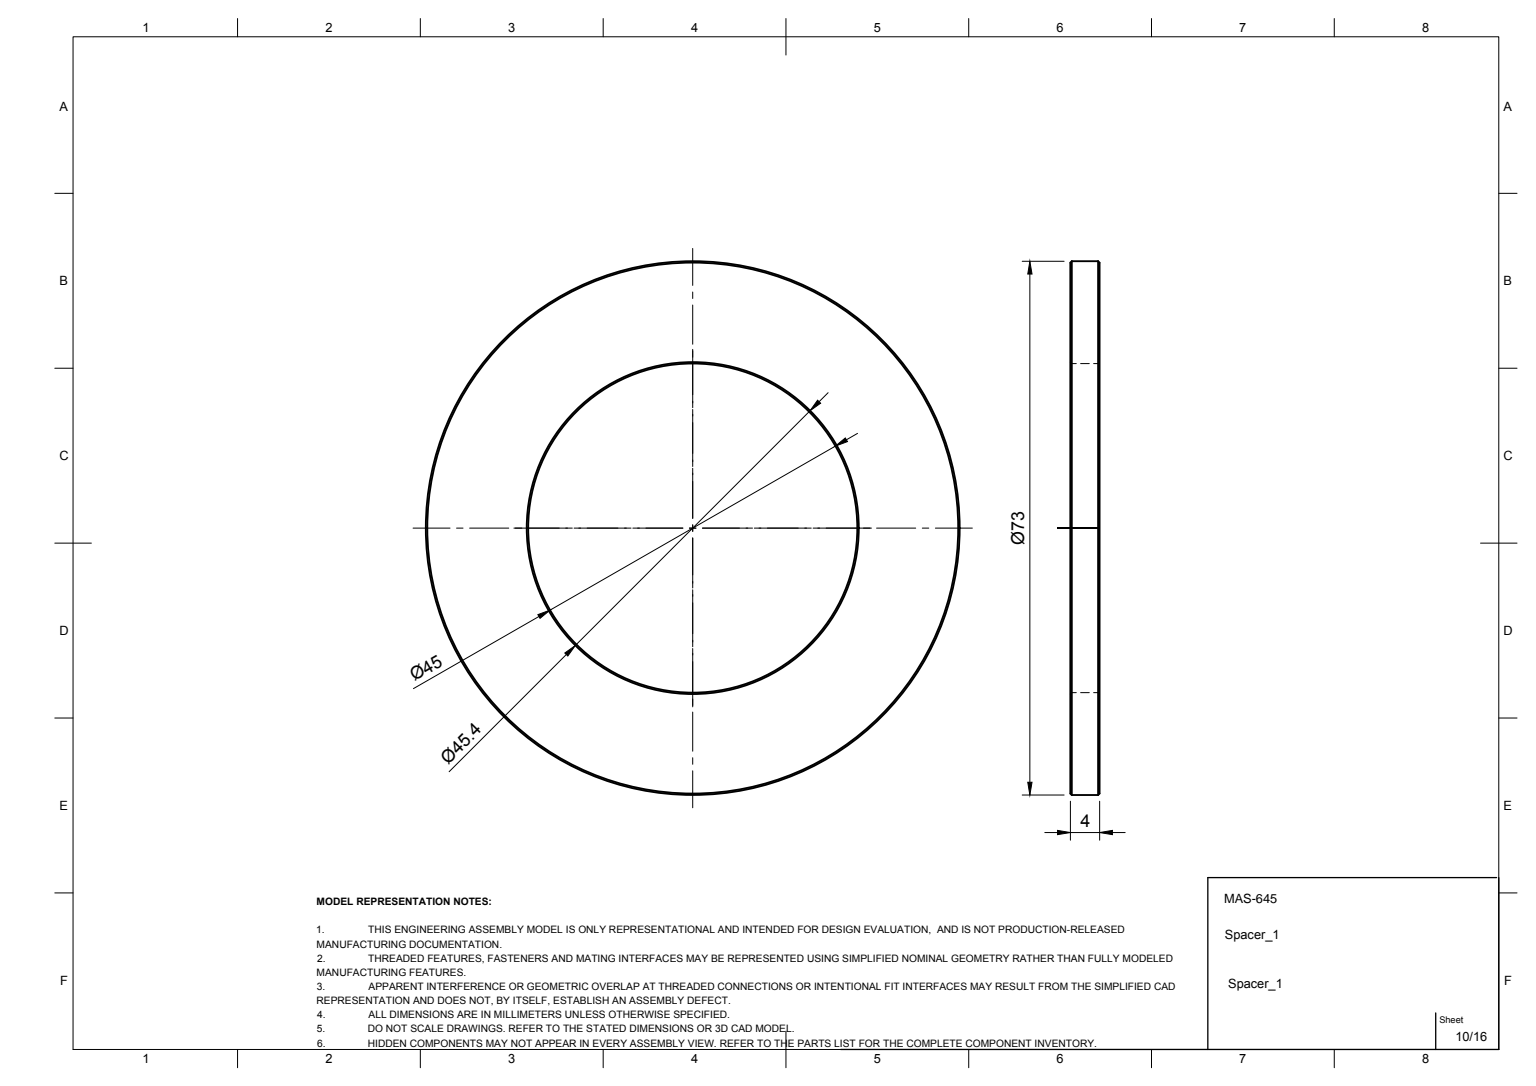
ISO-10303-21;
HEADER;
FILE_DESCRIPTION((''),'2;1');
FILE_NAME('Spacer_1.step','2026-10-09T10:54:55-07:00',(''),(''),'','','');
FILE_SCHEMA (('AUTOMOTIVE_DESIGN { 1 0 10303 214 3 1 1 }'));
ENDSEC;
DATA;
#10=MECHANICAL_DESIGN_GEOMETRIC_PRESENTATION_REPRESENTATION('',(#607),#63824);
#577=SHAPE_REPRESENTATION_RELATIONSHIP('SRR','None',#63891,#592) ;
#592=ADVANCED_BREP_SHAPE_REPRESENTATION('',(#622),#63821) ;
#607=STYLED_ITEM('',(#63963),#622) ;
#622=MANIFOLD_SOLID_BREP('Body1',#15506) ;
#794=FACE_BOUND('',#3406,.T.) ;
#795=FACE_BOUND('',#3412,.T.) ;
#1110=PLANE('',#17806) ;
#1111=PLANE('',#17816) ;
#1523=CYLINDRICAL_SURFACE('',#17808,36.5) ;
#1524=CYLINDRICAL_SURFACE('',#17812,22.5) ;
#2374=FACE_OUTER_BOUND('',#3404,.T.) ;
#2375=FACE_OUTER_BOUND('',#3405,.T.) ;
#2376=FACE_OUTER_BOUND('',#3407,.T.) ;
#2377=FACE_OUTER_BOUND('',#3408,.T.) ;
#2378=FACE_OUTER_BOUND('',#3409,.T.) ;
#2379=FACE_OUTER_BOUND('',#3410,.T.) ;
#2380=FACE_OUTER_BOUND('',#3411,.T.) ;
#2381=FACE_OUTER_BOUND('',#3413,.T.) ;
#3404=EDGE_LOOP('',(#14348,#14349,#14350,#14351)) ;
#3405=EDGE_LOOP('',(#14352)) ;
#3406=EDGE_LOOP('',(#14353)) ;
#3407=EDGE_LOOP('',(#14354,#14355,#14356,#14357)) ;
#3408=EDGE_LOOP('',(#14358,#14359,#14360,#14361)) ;
#3409=EDGE_LOOP('',(#14362,#14363,#14364,#14365)) ;
#3410=EDGE_LOOP('',(#14366,#14367,#14368,#14369)) ;
#3411=EDGE_LOOP('',(#14370)) ;
#3412=EDGE_LOOP('',(#14371)) ;
#3413=EDGE_LOOP('',(#14372,#14373,#14374,#14375)) ;
#4642=CIRCLE('',#17804,36.5) ;
#4643=CIRCLE('',#17805,36.3) ;
#4644=CIRCLE('',#17807,22.7) ;
#4645=CIRCLE('',#17809,36.5) ;
#4646=CIRCLE('',#17811,22.5) ;
#4647=CIRCLE('',#17813,22.5) ;
#4648=CIRCLE('',#17815,36.3) ;
#4649=CIRCLE('',#17817,22.7) ;
#5320=LINE('',#63622,#5976) ;
#5321=LINE('',#63630,#5977) ;
#5322=LINE('',#63634,#5978) ;
#5323=LINE('',#63637,#5979) ;
#5324=LINE('',#63641,#5980) ;
#5325=LINE('',#63647,#5981) ;
#5976=VECTOR('',#22792,36.4) ;
#5977=VECTOR('',#22803,36.5) ;
#5978=VECTOR('',#22808,22.6) ;
#5979=VECTOR('',#22811,22.5) ;
#5980=VECTOR('',#22816,36.4) ;
#5981=VECTOR('',#22825,22.6) ;
#7407=VERTEX_POINT('',#63619) ;
#7408=VERTEX_POINT('',#63621) ;
#7409=VERTEX_POINT('',#63625) ;
#7410=VERTEX_POINT('',#63628) ;
#7411=VERTEX_POINT('',#63632) ;
#7412=VERTEX_POINT('',#63636) ;
#7413=VERTEX_POINT('',#63640) ;
#7414=VERTEX_POINT('',#63644) ;
#9728=EDGE_CURVE('',#7407,#7407,#4642,.T.) ;
#9729=EDGE_CURVE('',#7407,#7408,#5320,.T.) ;
#9730=EDGE_CURVE('',#7408,#7408,#4643,.T.) ;
#9731=EDGE_CURVE('',#7409,#7409,#4644,.T.) ;
#9732=EDGE_CURVE('',#7410,#7410,#4645,.T.) ;
#9733=EDGE_CURVE('',#7410,#7407,#5321,.T.) ;
#9734=EDGE_CURVE('',#7411,#7411,#4646,.T.) ;
#9735=EDGE_CURVE('',#7411,#7409,#5322,.T.) ;
#9736=EDGE_CURVE('',#7411,#7412,#5323,.T.) ;
#9737=EDGE_CURVE('',#7412,#7412,#4647,.T.) ;
#9738=EDGE_CURVE('',#7410,#7413,#5324,.T.) ;
#9739=EDGE_CURVE('',#7413,#7413,#4648,.T.) ;
#9740=EDGE_CURVE('',#7414,#7414,#4649,.T.) ;
#9741=EDGE_CURVE('',#7412,#7414,#5325,.T.) ;
#14348=ORIENTED_EDGE('',*,*,#9728,.T.) ;
#14349=ORIENTED_EDGE('',*,*,#9729,.T.) ;
#14350=ORIENTED_EDGE('',*,*,#9730,.T.) ;
#14351=ORIENTED_EDGE('',*,*,#9729,.F.) ;
#14352=ORIENTED_EDGE('',*,*,#9730,.F.) ;
#14353=ORIENTED_EDGE('',*,*,#9731,.F.) ;
#14354=ORIENTED_EDGE('',*,*,#9732,.F.) ;
#14355=ORIENTED_EDGE('',*,*,#9733,.T.) ;
#14356=ORIENTED_EDGE('',*,*,#9728,.F.) ;
#14357=ORIENTED_EDGE('',*,*,#9733,.F.) ;
#14358=ORIENTED_EDGE('',*,*,#9734,.T.) ;
#14359=ORIENTED_EDGE('',*,*,#9735,.T.) ;
#14360=ORIENTED_EDGE('',*,*,#9731,.T.) ;
#14361=ORIENTED_EDGE('',*,*,#9735,.F.) ;
#14362=ORIENTED_EDGE('',*,*,#9734,.F.) ;
#14363=ORIENTED_EDGE('',*,*,#9736,.T.) ;
#14364=ORIENTED_EDGE('',*,*,#9737,.F.) ;
#14365=ORIENTED_EDGE('',*,*,#9736,.F.) ;
#14366=ORIENTED_EDGE('',*,*,#9732,.T.) ;
#14367=ORIENTED_EDGE('',*,*,#9738,.T.) ;
#14368=ORIENTED_EDGE('',*,*,#9739,.T.) ;
#14369=ORIENTED_EDGE('',*,*,#9738,.F.) ;
#14370=ORIENTED_EDGE('',*,*,#9739,.F.) ;
#14371=ORIENTED_EDGE('',*,*,#9740,.F.) ;
#14372=ORIENTED_EDGE('',*,*,#9737,.T.) ;
#14373=ORIENTED_EDGE('',*,*,#9741,.T.) ;
#14374=ORIENTED_EDGE('',*,*,#9740,.T.) ;
#14375=ORIENTED_EDGE('',*,*,#9741,.F.) ;
#14629=CONICAL_SURFACE('',#17803,36.4,0.785398163397449) ;
#14630=CONICAL_SURFACE('',#17810,22.6,0.785398163397449) ;
#14631=CONICAL_SURFACE('',#17814,36.4,0.785398163397448) ;
#14632=CONICAL_SURFACE('',#17818,22.6,0.785398163397448) ;
#15462=ADVANCED_FACE('',(#2374),#14629,.T.) ;
#15463=ADVANCED_FACE('',(#2375,#794),#1110,.F.) ;
#15464=ADVANCED_FACE('',(#2376),#1523,.T.) ;
#15465=ADVANCED_FACE('',(#2377),#14630,.F.) ;
#15466=ADVANCED_FACE('',(#2378),#1524,.F.) ;
#15467=ADVANCED_FACE('',(#2379),#14631,.T.) ;
#15468=ADVANCED_FACE('',(#2380,#795),#1111,.T.) ;
#15469=ADVANCED_FACE('',(#2381),#14632,.F.) ;
#15506=CLOSED_SHELL('',(#15462,#15463,#15464,#15465,#15466,#15467,#15468,
#15469)) ;
#17802=AXIS2_PLACEMENT_3D('',#63617,#22786,#22787) ;
#17803=AXIS2_PLACEMENT_3D('',#63618,#22788,#22789) ;
#17804=AXIS2_PLACEMENT_3D('',#63620,#22790,#22791) ;
#17805=AXIS2_PLACEMENT_3D('',#63623,#22793,#22794) ;
#17806=AXIS2_PLACEMENT_3D('',#63624,#22795,#22796) ;
#17807=AXIS2_PLACEMENT_3D('',#63626,#22797,#22798) ;
#17808=AXIS2_PLACEMENT_3D('',#63627,#22799,#22800) ;
#17809=AXIS2_PLACEMENT_3D('',#63629,#22801,#22802) ;
#17810=AXIS2_PLACEMENT_3D('',#63631,#22804,#22805) ;
#17811=AXIS2_PLACEMENT_3D('',#63633,#22806,#22807) ;
#17812=AXIS2_PLACEMENT_3D('',#63635,#22809,#22810) ;
#17813=AXIS2_PLACEMENT_3D('',#63638,#22812,#22813) ;
#17814=AXIS2_PLACEMENT_3D('',#63639,#22814,#22815) ;
#17815=AXIS2_PLACEMENT_3D('',#63642,#22817,#22818) ;
#17816=AXIS2_PLACEMENT_3D('',#63643,#22819,#22820) ;
#17817=AXIS2_PLACEMENT_3D('',#63645,#22821,#22822) ;
#17818=AXIS2_PLACEMENT_3D('',#63646,#22823,#22824) ;
#22786=DIRECTION('axis',(0.,0.,1.)) ;
#22787=DIRECTION('refdir',(1.,0.,0.)) ;
#22788=DIRECTION('center_axis',(0.,0.,1.)) ;
#22789=DIRECTION('ref_axis',(1.,0.,0.)) ;
#22790=DIRECTION('center_axis',(0.,0.,-1.)) ;
#22791=DIRECTION('ref_axis',(1.,0.,0.)) ;
#22792=DIRECTION('',(0.707106781186548,8.65956056235494E-17,-0.707106781186547)) ;
#22793=DIRECTION('center_axis',(0.,0.,1.)) ;
#22794=DIRECTION('ref_axis',(1.,0.,0.)) ;
#22795=DIRECTION('center_axis',(0.,0.,1.)) ;
#22796=DIRECTION('ref_axis',(1.,0.,0.)) ;
#22797=DIRECTION('center_axis',(0.,0.,-1.)) ;
#22798=DIRECTION('ref_axis',(1.,0.,0.)) ;
#22799=DIRECTION('center_axis',(0.,0.,1.)) ;
#22800=DIRECTION('ref_axis',(1.,0.,0.)) ;
#22801=DIRECTION('center_axis',(0.,0.,1.)) ;
#22802=DIRECTION('ref_axis',(1.,0.,0.)) ;
#22803=DIRECTION('',(0.,0.,-1.)) ;
#22804=DIRECTION('center_axis',(0.,0.,-1.)) ;
#22805=DIRECTION('ref_axis',(1.,0.,0.)) ;
#22806=DIRECTION('center_axis',(0.,0.,1.)) ;
#22807=DIRECTION('ref_axis',(1.,0.,0.)) ;
#22808=DIRECTION('',(-0.707106781186548,8.65956056235494E-17,-0.707106781186547)) ;
#22809=DIRECTION('center_axis',(0.,0.,1.)) ;
#22810=DIRECTION('ref_axis',(1.,0.,0.)) ;
#22811=DIRECTION('',(0.,0.,1.)) ;
#22812=DIRECTION('center_axis',(0.,0.,-1.)) ;
#22813=DIRECTION('ref_axis',(1.,0.,0.)) ;
#22814=DIRECTION('center_axis',(0.,0.,-1.)) ;
#22815=DIRECTION('ref_axis',(1.,0.,0.)) ;
#22816=DIRECTION('',(0.707106781186547,-8.65956056235493E-17,0.707106781186548)) ;
#22817=DIRECTION('center_axis',(0.,0.,-1.)) ;
#22818=DIRECTION('ref_axis',(1.,0.,0.)) ;
#22819=DIRECTION('center_axis',(0.,0.,1.)) ;
#22820=DIRECTION('ref_axis',(1.,0.,0.)) ;
#22821=DIRECTION('center_axis',(0.,0.,1.)) ;
#22822=DIRECTION('ref_axis',(1.,0.,0.)) ;
#22823=DIRECTION('center_axis',(0.,0.,1.)) ;
#22824=DIRECTION('ref_axis',(1.,0.,0.)) ;
#22825=DIRECTION('',(-0.707106781186547,-8.65956056235493E-17,0.707106781186548)) ;
#63617=CARTESIAN_POINT('',(0.,0.,0.)) ;
#63618=CARTESIAN_POINT('Origin',(0.,0.,0.1)) ;
#63619=CARTESIAN_POINT('',(-36.5,4.46996081688784E-15,0.2)) ;
#63620=CARTESIAN_POINT('Origin',(0.,0.,0.2)) ;
#63621=CARTESIAN_POINT('',(-36.3,-4.44546788090489E-15,0.)) ;
#63622=CARTESIAN_POINT('',(-36.4,-4.45771434889637E-15,0.1)) ;
#63623=CARTESIAN_POINT('Origin',(0.,0.,0.)) ;
#63624=CARTESIAN_POINT('Origin',(0.,0.,0.)) ;
#63625=CARTESIAN_POINT('',(-22.7,2.77994823406449E-15,0.)) ;
#63626=CARTESIAN_POINT('Origin',(0.,0.,0.)) ;
#63627=CARTESIAN_POINT('Origin',(0.,0.,0.)) ;
#63628=CARTESIAN_POINT('',(-36.5,-4.46996081688784E-15,3.8)) ;
#63629=CARTESIAN_POINT('Origin',(0.,0.,3.8)) ;
#63630=CARTESIAN_POINT('',(-36.5,-4.46996081688784E-15,0.)) ;
#63631=CARTESIAN_POINT('Origin',(0.,0.,0.1)) ;
#63632=CARTESIAN_POINT('',(-22.5,-2.75545529808154E-15,0.2)) ;
#63633=CARTESIAN_POINT('Origin',(0.,0.,0.2)) ;
#63634=CARTESIAN_POINT('',(-22.6,2.76770176607302E-15,0.1)) ;
#63635=CARTESIAN_POINT('Origin',(0.,0.,0.)) ;
#63636=CARTESIAN_POINT('',(-22.5,2.75545529808154E-15,3.8)) ;
#63637=CARTESIAN_POINT('',(-22.5,-2.75545529808154E-15,0.)) ;
#63638=CARTESIAN_POINT('Origin',(0.,0.,3.8)) ;
#63639=CARTESIAN_POINT('Origin',(0.,0.,3.9)) ;
#63640=CARTESIAN_POINT('',(-36.3,4.44546788090489E-15,4.)) ;
#63641=CARTESIAN_POINT('',(-36.4,4.45771434889637E-15,3.9)) ;
#63642=CARTESIAN_POINT('Origin',(0.,0.,4.)) ;
#63643=CARTESIAN_POINT('Origin',(0.,0.,4.)) ;
#63644=CARTESIAN_POINT('',(-22.7,-2.77994823406449E-15,4.)) ;
#63645=CARTESIAN_POINT('Origin',(0.,0.,4.)) ;
#63646=CARTESIAN_POINT('Origin',(0.,0.,3.9)) ;
#63647=CARTESIAN_POINT('',(-22.6,-2.76770176607302E-15,3.9)) ;
#63804=UNCERTAINTY_MEASURE_WITH_UNIT(LENGTH_MEASURE(0.01),#63825,
'DISTANCE_ACCURACY_VALUE',
'Maximum model space distance between geometric entities at asserted c
onnectivities') ;
#63807=UNCERTAINTY_MEASURE_WITH_UNIT(LENGTH_MEASURE(0.01),#63825,
'DISTANCE_ACCURACY_VALUE',
'Maximum model space distance between geometric entities at asserted c
onnectivities') ;
#63821=(
GEOMETRIC_REPRESENTATION_CONTEXT(3)
GLOBAL_UNCERTAINTY_ASSIGNED_CONTEXT((#63804))
GLOBAL_UNIT_ASSIGNED_CONTEXT((#63825,#63827,#63828))
REPRESENTATION_CONTEXT('','3D')
) ;
#63824=(
GEOMETRIC_REPRESENTATION_CONTEXT(3)
GLOBAL_UNCERTAINTY_ASSIGNED_CONTEXT((#63807))
GLOBAL_UNIT_ASSIGNED_CONTEXT((#63825,#63827,#63828))
REPRESENTATION_CONTEXT('','3D')
) ;
#63825=(
LENGTH_UNIT()
NAMED_UNIT(*)
SI_UNIT(.MILLI.,.METRE.)
) ;
#63827=(
NAMED_UNIT(*)
PLANE_ANGLE_UNIT()
SI_UNIT($,.RADIAN.)
) ;
#63828=(
NAMED_UNIT(*)
SI_UNIT($,.STERADIAN.)
SOLID_ANGLE_UNIT()
) ;
#63842=SHAPE_DEFINITION_REPRESENTATION(#63858,#63891) ;
#63858=PRODUCT_DEFINITION_SHAPE('',$,#63908) ;
#63891=SHAPE_REPRESENTATION('',(#17802),#63821) ;
#63894=PRODUCT_DEFINITION_CONTEXT('part definition',#63944,'design') ;
#63908=PRODUCT_DEFINITION('Spacer_1','Spacer_1',#63924,#63894) ;
#63924=PRODUCT_DEFINITION_FORMATION('',$,#63959) ;
#63944=APPLICATION_CONTEXT(
'Core Data for Automotive Mechanical Design Process') ;
#63945=PRODUCT_CONTEXT('part definition',#63944,'mechanical') ;
#63959=PRODUCT('Spacer_1','Spacer_1',$,(#63945)) ;
#63963=PRESENTATION_STYLE_ASSIGNMENT((#63968)) ;
#63968=SURFACE_STYLE_USAGE(.BOTH.,#63973) ;
#63973=SURFACE_SIDE_STYLE('',(#63978)) ;
#63978=SURFACE_STYLE_FILL_AREA(#63983) ;
#63983=FILL_AREA_STYLE('Opaque(160,160,160)',(#63988)) ;
#63988=FILL_AREA_STYLE_COLOUR('Opaque(160,160,160)',#63993) ;
#63993=COLOUR_RGB('Opaque(160,160,160)', 0.09019608, 0.27058824, 0.51372549) ;
ENDSEC;
END-ISO-10303-21;
